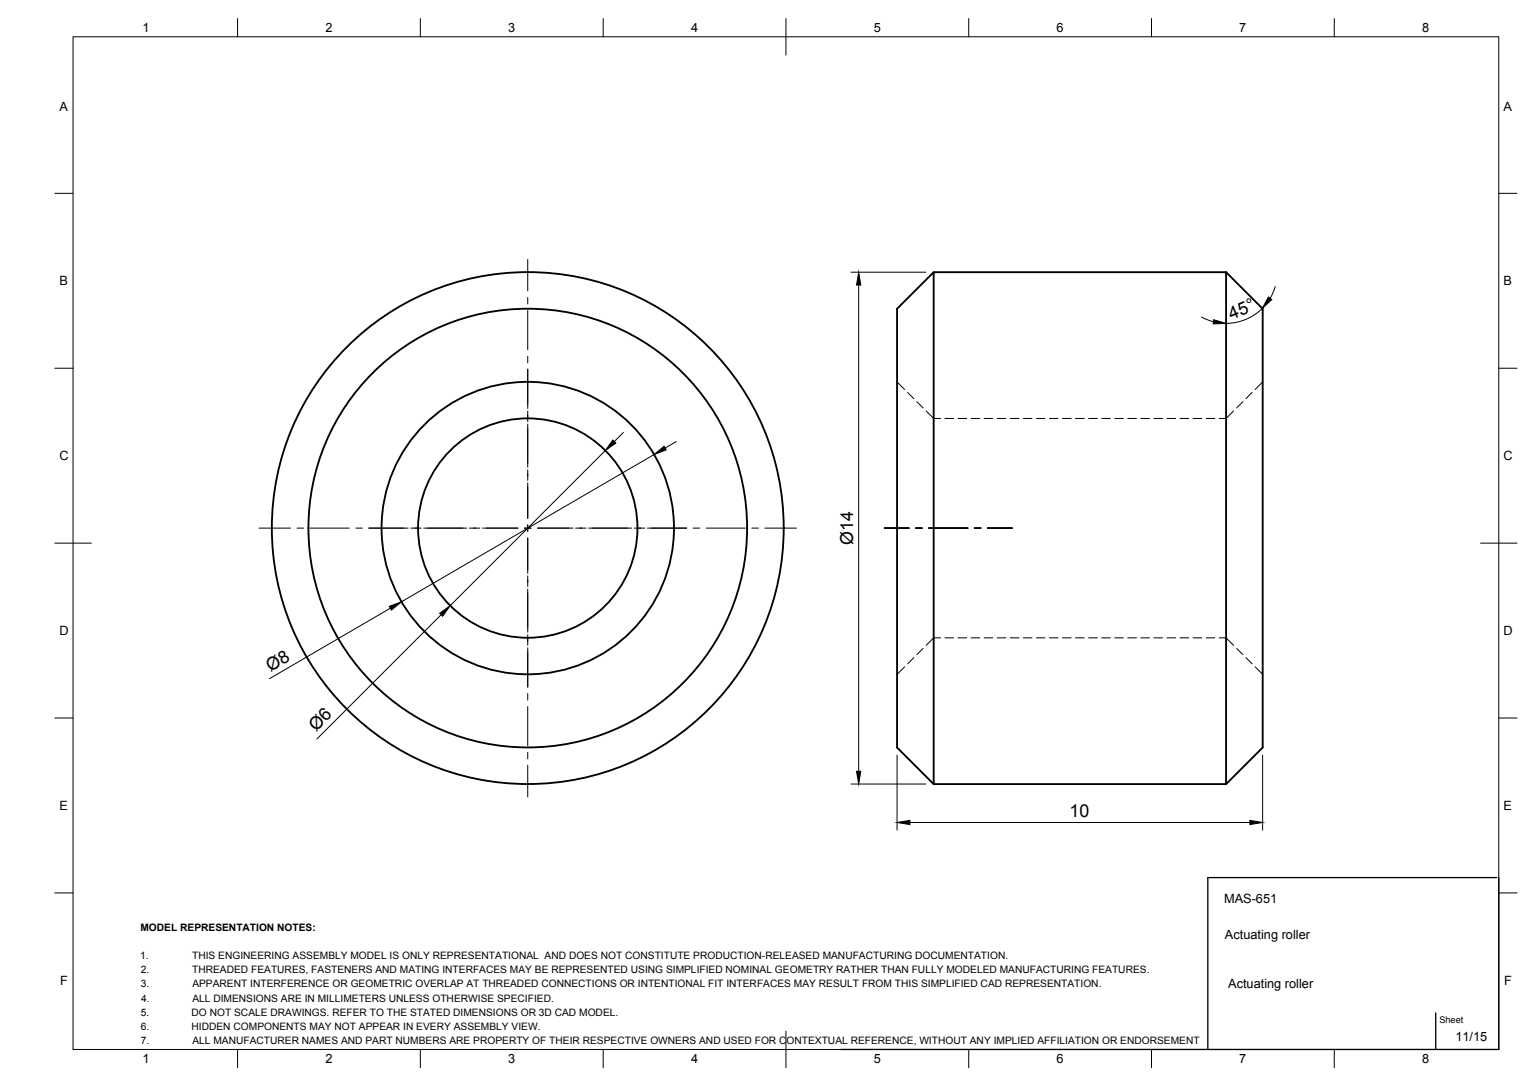
ISO-10303-21;
HEADER;
/* Generated by software containing ST-Developer
 * from STEP Tools, Inc. (www.steptools.com) 
 */

FILE_DESCRIPTION(
/* description */ ('Independent direct-acting normally-closed roller-plunger limit-switch
 CAD. Removable cover, insulated terminal supports, captured bus/conta
ct bridge, native Coil return spring, integral lower travel stop, reus
able instanced hardware and free roller. Manual geometric contact open
ing4mm; no snap-action/contact-force, electrical/current/voltage, envi
ronmental seal, safety-switch, wear, load or life certification. Exter
nal wiring and anchors omitted; fits and application engineering requi
red.'),
/* implementation_level */ '2;1');

FILE_NAME(
/* name */ 'Actuating roller.step',
/* time_stamp */ '2026-11-08T07:32:43-08:00',
/* author */ (''),
/* organization */ (''),
/* preprocessor_version */ 'ST-DEVELOPER v20.2',
/* originating_system */ 'Autodesk Translation Framework v15.17.0.0',
/* authorisation */ '');

FILE_SCHEMA (('AUTOMOTIVE_DESIGN { 1 0 10303 214 3 1 1 }'));
ENDSEC;

DATA;
#10=MECHANICAL_DESIGN_GEOMETRIC_PRESENTATION_REPRESENTATION('',(#181),#36482);
#135=CONICAL_SURFACE('',#10298,0.65,0.785398163397448);
#136=CONICAL_SURFACE('',#10305,0.65,0.785398163397448);
#137=CONICAL_SURFACE('',#10309,0.35,0.785398163397448);
#138=CONICAL_SURFACE('',#10313,0.35,0.785398163397448);
#147=SHAPE_REPRESENTATION_RELATIONSHIP('SRR','None',#36560,#164);
#164=ADVANCED_BREP_SHAPE_REPRESENTATION('',(#198),#36470);
#181=STYLED_ITEM('',(#36654),#198);
#198=MANIFOLD_SOLID_BREP('Roller',#9772);
#280=FACE_BOUND('',#1272,.T.);
#281=FACE_BOUND('',#1275,.T.);
#366=PLANE('',#10303);
#367=PLANE('',#10307);
#686=FACE_OUTER_BOUND('',#1269,.T.);
#687=FACE_OUTER_BOUND('',#1270,.T.);
#688=FACE_OUTER_BOUND('',#1271,.T.);
#689=FACE_OUTER_BOUND('',#1273,.T.);
#690=FACE_OUTER_BOUND('',#1274,.T.);
#691=FACE_OUTER_BOUND('',#1276,.T.);
#692=FACE_OUTER_BOUND('',#1277,.T.);
#693=FACE_OUTER_BOUND('',#1278,.T.);
#1269=EDGE_LOOP('',(#7338,#7339,#7340,#7341));
#1270=EDGE_LOOP('',(#7342,#7343,#7344,#7345));
#1271=EDGE_LOOP('',(#7346));
#1272=EDGE_LOOP('',(#7347));
#1273=EDGE_LOOP('',(#7348,#7349,#7350,#7351));
#1274=EDGE_LOOP('',(#7352));
#1275=EDGE_LOOP('',(#7353));
#1276=EDGE_LOOP('',(#7354,#7355,#7356,#7357));
#1277=EDGE_LOOP('',(#7358,#7359,#7360,#7361));
#1278=EDGE_LOOP('',(#7362,#7363,#7364,#7365));
#1666=CIRCLE('',#10299,0.7);
#1667=CIRCLE('',#10300,0.6);
#1668=CIRCLE('',#10302,0.7);
#1669=CIRCLE('',#10304,0.4);
#1670=CIRCLE('',#10306,0.6);
#1671=CIRCLE('',#10308,0.4);
#1672=CIRCLE('',#10310,0.3);
#1673=CIRCLE('',#10312,0.3);
#2721=LINE('',#23180,#3295);
#2722=LINE('',#23185,#3296);
#2723=LINE('',#23192,#3297);
#2724=LINE('',#23199,#3298);
#2725=LINE('',#23203,#3299);
#2726=LINE('',#23205,#3300);
#3295=VECTOR('',#11622,0.65);
#3296=VECTOR('',#11629,0.7);
#3297=VECTOR('',#11638,0.65);
#3298=VECTOR('',#11647,0.35);
#3299=VECTOR('',#11652,0.3);
#3300=VECTOR('',#11655,0.35);
#4043=VERTEX_POINT('',#23177);
#4044=VERTEX_POINT('',#23179);
#4045=VERTEX_POINT('',#23183);
#4046=VERTEX_POINT('',#23187);
#4047=VERTEX_POINT('',#23190);
#4048=VERTEX_POINT('',#23194);
#4049=VERTEX_POINT('',#23197);
#4050=VERTEX_POINT('',#23201);
#5225=EDGE_CURVE('',#4043,#4043,#1666,.T.);
#5226=EDGE_CURVE('',#4043,#4044,#2721,.T.);
#5227=EDGE_CURVE('',#4044,#4044,#1667,.T.);
#5228=EDGE_CURVE('',#4045,#4045,#1668,.T.);
#5229=EDGE_CURVE('',#4045,#4043,#2722,.T.);
#5230=EDGE_CURVE('',#4046,#4046,#1669,.T.);
#5231=EDGE_CURVE('',#4047,#4047,#1670,.T.);
#5232=EDGE_CURVE('',#4047,#4045,#2723,.T.);
#5233=EDGE_CURVE('',#4048,#4048,#1671,.T.);
#5234=EDGE_CURVE('',#4049,#4049,#1672,.T.);
#5235=EDGE_CURVE('',#4049,#4046,#2724,.T.);
#5236=EDGE_CURVE('',#4050,#4050,#1673,.T.);
#5237=EDGE_CURVE('',#4050,#4049,#2725,.T.);
#5238=EDGE_CURVE('',#4048,#4050,#2726,.T.);
#7338=ORIENTED_EDGE('',*,*,#5225,.T.);
#7339=ORIENTED_EDGE('',*,*,#5226,.T.);
#7340=ORIENTED_EDGE('',*,*,#5227,.T.);
#7341=ORIENTED_EDGE('',*,*,#5226,.F.);
#7342=ORIENTED_EDGE('',*,*,#5228,.F.);
#7343=ORIENTED_EDGE('',*,*,#5229,.T.);
#7344=ORIENTED_EDGE('',*,*,#5225,.F.);
#7345=ORIENTED_EDGE('',*,*,#5229,.F.);
#7346=ORIENTED_EDGE('',*,*,#5227,.F.);
#7347=ORIENTED_EDGE('',*,*,#5230,.F.);
#7348=ORIENTED_EDGE('',*,*,#5231,.T.);
#7349=ORIENTED_EDGE('',*,*,#5232,.T.);
#7350=ORIENTED_EDGE('',*,*,#5228,.T.);
#7351=ORIENTED_EDGE('',*,*,#5232,.F.);
#7352=ORIENTED_EDGE('',*,*,#5231,.F.);
#7353=ORIENTED_EDGE('',*,*,#5233,.F.);
#7354=ORIENTED_EDGE('',*,*,#5234,.T.);
#7355=ORIENTED_EDGE('',*,*,#5235,.T.);
#7356=ORIENTED_EDGE('',*,*,#5230,.T.);
#7357=ORIENTED_EDGE('',*,*,#5235,.F.);
#7358=ORIENTED_EDGE('',*,*,#5236,.F.);
#7359=ORIENTED_EDGE('',*,*,#5237,.T.);
#7360=ORIENTED_EDGE('',*,*,#5234,.F.);
#7361=ORIENTED_EDGE('',*,*,#5237,.F.);
#7362=ORIENTED_EDGE('',*,*,#5233,.T.);
#7363=ORIENTED_EDGE('',*,*,#5238,.T.);
#7364=ORIENTED_EDGE('',*,*,#5236,.T.);
#7365=ORIENTED_EDGE('',*,*,#5238,.F.);
#9031=CYLINDRICAL_SURFACE('',#10301,0.7);
#9032=CYLINDRICAL_SURFACE('',#10311,0.3);
#9476=ADVANCED_FACE('',(#686),#135,.T.);
#9477=ADVANCED_FACE('',(#687),#9031,.T.);
#9478=ADVANCED_FACE('',(#688,#280),#366,.F.);
#9479=ADVANCED_FACE('',(#689),#136,.T.);
#9480=ADVANCED_FACE('',(#690,#281),#367,.T.);
#9481=ADVANCED_FACE('',(#691),#137,.F.);
#9482=ADVANCED_FACE('',(#692),#9032,.F.);
#9483=ADVANCED_FACE('',(#693),#138,.F.);
#9772=CLOSED_SHELL('',(#9476,#9477,#9478,#9479,#9480,#9481,#9482,#9483));
#10297=AXIS2_PLACEMENT_3D('',#23175,#11616,#11617);
#10298=AXIS2_PLACEMENT_3D('',#23176,#11618,#11619);
#10299=AXIS2_PLACEMENT_3D('',#23178,#11620,#11621);
#10300=AXIS2_PLACEMENT_3D('',#23181,#11623,#11624);
#10301=AXIS2_PLACEMENT_3D('',#23182,#11625,#11626);
#10302=AXIS2_PLACEMENT_3D('',#23184,#11627,#11628);
#10303=AXIS2_PLACEMENT_3D('',#23186,#11630,#11631);
#10304=AXIS2_PLACEMENT_3D('',#23188,#11632,#11633);
#10305=AXIS2_PLACEMENT_3D('',#23189,#11634,#11635);
#10306=AXIS2_PLACEMENT_3D('',#23191,#11636,#11637);
#10307=AXIS2_PLACEMENT_3D('',#23193,#11639,#11640);
#10308=AXIS2_PLACEMENT_3D('',#23195,#11641,#11642);
#10309=AXIS2_PLACEMENT_3D('',#23196,#11643,#11644);
#10310=AXIS2_PLACEMENT_3D('',#23198,#11645,#11646);
#10311=AXIS2_PLACEMENT_3D('',#23200,#11648,#11649);
#10312=AXIS2_PLACEMENT_3D('',#23202,#11650,#11651);
#10313=AXIS2_PLACEMENT_3D('',#23204,#11653,#11654);
#11616=DIRECTION('axis',(0.,0.,1.));
#11617=DIRECTION('refdir',(1.,0.,0.));
#11618=DIRECTION('center_axis',(0.,0.,1.));
#11619=DIRECTION('ref_axis',(1.,0.,0.));
#11620=DIRECTION('center_axis',(0.,0.,-1.));
#11621=DIRECTION('ref_axis',(1.,0.,0.));
#11622=DIRECTION('',(0.707106781186547,8.65956056235493E-17,-0.707106781186548));
#11623=DIRECTION('center_axis',(0.,0.,1.));
#11624=DIRECTION('ref_axis',(1.,0.,0.));
#11625=DIRECTION('center_axis',(0.,0.,1.));
#11626=DIRECTION('ref_axis',(1.,0.,0.));
#11627=DIRECTION('center_axis',(0.,0.,1.));
#11628=DIRECTION('ref_axis',(1.,0.,0.));
#11629=DIRECTION('',(0.,0.,-1.));
#11630=DIRECTION('center_axis',(0.,0.,1.));
#11631=DIRECTION('ref_axis',(1.,0.,0.));
#11632=DIRECTION('center_axis',(0.,0.,-1.));
#11633=DIRECTION('ref_axis',(1.,0.,0.));
#11634=DIRECTION('center_axis',(0.,0.,-1.));
#11635=DIRECTION('ref_axis',(1.,0.,0.));
#11636=DIRECTION('center_axis',(0.,0.,-1.));
#11637=DIRECTION('ref_axis',(1.,0.,0.));
#11638=DIRECTION('',(-0.707106781186548,-8.65956056235494E-17,-0.707106781186548));
#11639=DIRECTION('center_axis',(0.,0.,1.));
#11640=DIRECTION('ref_axis',(1.,0.,0.));
#11641=DIRECTION('center_axis',(0.,0.,1.));
#11642=DIRECTION('ref_axis',(1.,0.,0.));
#11643=DIRECTION('center_axis',(0.,0.,-1.));
#11644=DIRECTION('ref_axis',(1.,0.,0.));
#11645=DIRECTION('center_axis',(0.,0.,1.));
#11646=DIRECTION('ref_axis',(1.,0.,0.));
#11647=DIRECTION('',(-0.707106781186547,-8.65956056235493E-17,-0.707106781186548));
#11648=DIRECTION('center_axis',(0.,0.,1.));
#11649=DIRECTION('ref_axis',(1.,0.,0.));
#11650=DIRECTION('center_axis',(0.,0.,-1.));
#11651=DIRECTION('ref_axis',(1.,0.,0.));
#11652=DIRECTION('',(0.,0.,-1.));
#11653=DIRECTION('center_axis',(0.,0.,1.));
#11654=DIRECTION('ref_axis',(1.,0.,0.));
#11655=DIRECTION('',(0.707106781186547,8.65956056235493E-17,-0.707106781186547));
#23175=CARTESIAN_POINT('',(0.,0.,0.));
#23176=CARTESIAN_POINT('Origin',(0.,0.,0.05));
#23177=CARTESIAN_POINT('',(-0.7,8.57252759403147E-17,0.1));
#23178=CARTESIAN_POINT('Origin',(0.,0.,0.1));
#23179=CARTESIAN_POINT('',(-0.6,-7.34788079488412E-17,0.));
#23180=CARTESIAN_POINT('',(-0.65,-7.9602041944578E-17,0.05));
#23181=CARTESIAN_POINT('Origin',(0.,0.,0.));
#23182=CARTESIAN_POINT('Origin',(0.,0.,0.));
#23183=CARTESIAN_POINT('',(-0.7,-8.57252759403147E-17,0.9));
#23184=CARTESIAN_POINT('Origin',(0.,0.,0.9));
#23185=CARTESIAN_POINT('',(-0.7,-8.57252759403147E-17,0.));
#23186=CARTESIAN_POINT('Origin',(0.,0.,0.));
#23187=CARTESIAN_POINT('',(-0.4,4.89858719658941E-17,0.));
#23188=CARTESIAN_POINT('Origin',(0.,0.,0.));
#23189=CARTESIAN_POINT('Origin',(0.,0.,0.95));
#23190=CARTESIAN_POINT('',(-0.6,7.34788079488412E-17,1.));
#23191=CARTESIAN_POINT('Origin',(0.,0.,1.));
#23192=CARTESIAN_POINT('',(-0.65,-7.9602041944578E-17,0.95));
#23193=CARTESIAN_POINT('Origin',(0.,0.,1.));
#23194=CARTESIAN_POINT('',(-0.4,-4.89858719658941E-17,1.));
#23195=CARTESIAN_POINT('Origin',(0.,0.,1.));
#23196=CARTESIAN_POINT('Origin',(0.,0.,0.05));
#23197=CARTESIAN_POINT('',(-0.3,-3.67394039744206E-17,0.1));
#23198=CARTESIAN_POINT('Origin',(0.,0.,0.1));
#23199=CARTESIAN_POINT('',(-0.35,-4.28626379701574E-17,0.05));
#23200=CARTESIAN_POINT('Origin',(0.,0.,0.));
#23201=CARTESIAN_POINT('',(-0.3,3.67394039744206E-17,0.9));
#23202=CARTESIAN_POINT('Origin',(0.,0.,0.9));
#23203=CARTESIAN_POINT('',(-0.3,-3.67394039744206E-17,0.));
#23204=CARTESIAN_POINT('Origin',(0.,0.,0.95));
#23205=CARTESIAN_POINT('',(-0.35,-4.28626379701574E-17,0.95));
#36451=UNCERTAINTY_MEASURE_WITH_UNIT(LENGTH_MEASURE(0.001),#36483,
'DISTANCE_ACCURACY_VALUE',
'Maximum model space distance between geometric entities at asserted c
onnectivities');
#36463=UNCERTAINTY_MEASURE_WITH_UNIT(LENGTH_MEASURE(0.001),#36483,
'DISTANCE_ACCURACY_VALUE',
'Maximum model space distance between geometric entities at asserted c
onnectivities');
#36470=(
GEOMETRIC_REPRESENTATION_CONTEXT(3)
GLOBAL_UNCERTAINTY_ASSIGNED_CONTEXT((#36451))
GLOBAL_UNIT_ASSIGNED_CONTEXT((#36483,#36485,#36486))
REPRESENTATION_CONTEXT('','3D')
);
#36482=(
GEOMETRIC_REPRESENTATION_CONTEXT(3)
GLOBAL_UNCERTAINTY_ASSIGNED_CONTEXT((#36463))
GLOBAL_UNIT_ASSIGNED_CONTEXT((#36483,#36485,#36486))
REPRESENTATION_CONTEXT('','3D')
);
#36483=(
LENGTH_UNIT()
NAMED_UNIT(*)
SI_UNIT(.CENTI.,.METRE.)
);
#36485=(
NAMED_UNIT(*)
PLANE_ANGLE_UNIT()
SI_UNIT($,.RADIAN.)
);
#36486=(
NAMED_UNIT(*)
SI_UNIT($,.STERADIAN.)
SOLID_ANGLE_UNIT()
);
#36493=SHAPE_DEFINITION_REPRESENTATION(#36511,#36560);
#36511=PRODUCT_DEFINITION_SHAPE('',$,#36579);
#36560=SHAPE_REPRESENTATION('',(#10297),#36470);
#36572=PRODUCT_DEFINITION_CONTEXT('part definition',#36628,'design');
#36579=PRODUCT_DEFINITION('Actuating roller','Actuating roller',#36597,
#36572);
#36597=PRODUCT_DEFINITION_FORMATION('',$,#36636);
#36628=APPLICATION_CONTEXT(
'Core Data for Automotive Mechanical Design Process');
#36629=PRODUCT_CONTEXT('part definition',#36628,'mechanical');
#36636=PRODUCT('Actuating roller','Actuating roller',
'Turn concentric OD and bore, face and chamfer. Nominal dimensions in 
mm. Fit limits to be assigned at assembly level.',(#36629));
#36654=PRESENTATION_STYLE_ASSIGNMENT((#36668));
#36668=SURFACE_STYLE_USAGE(.BOTH.,#36682);
#36682=SURFACE_SIDE_STYLE('',(#36696));
#36696=SURFACE_STYLE_FILL_AREA(#36710);
#36710=FILL_AREA_STYLE('Roller gray',(#36724));
#36724=FILL_AREA_STYLE_COLOUR('Roller gray',#36738);
#36738=COLOUR_RGB('Roller gray',0.407843137254902,0.447058823529412,0.498039215686275);
ENDSEC;
END-ISO-10303-21;
